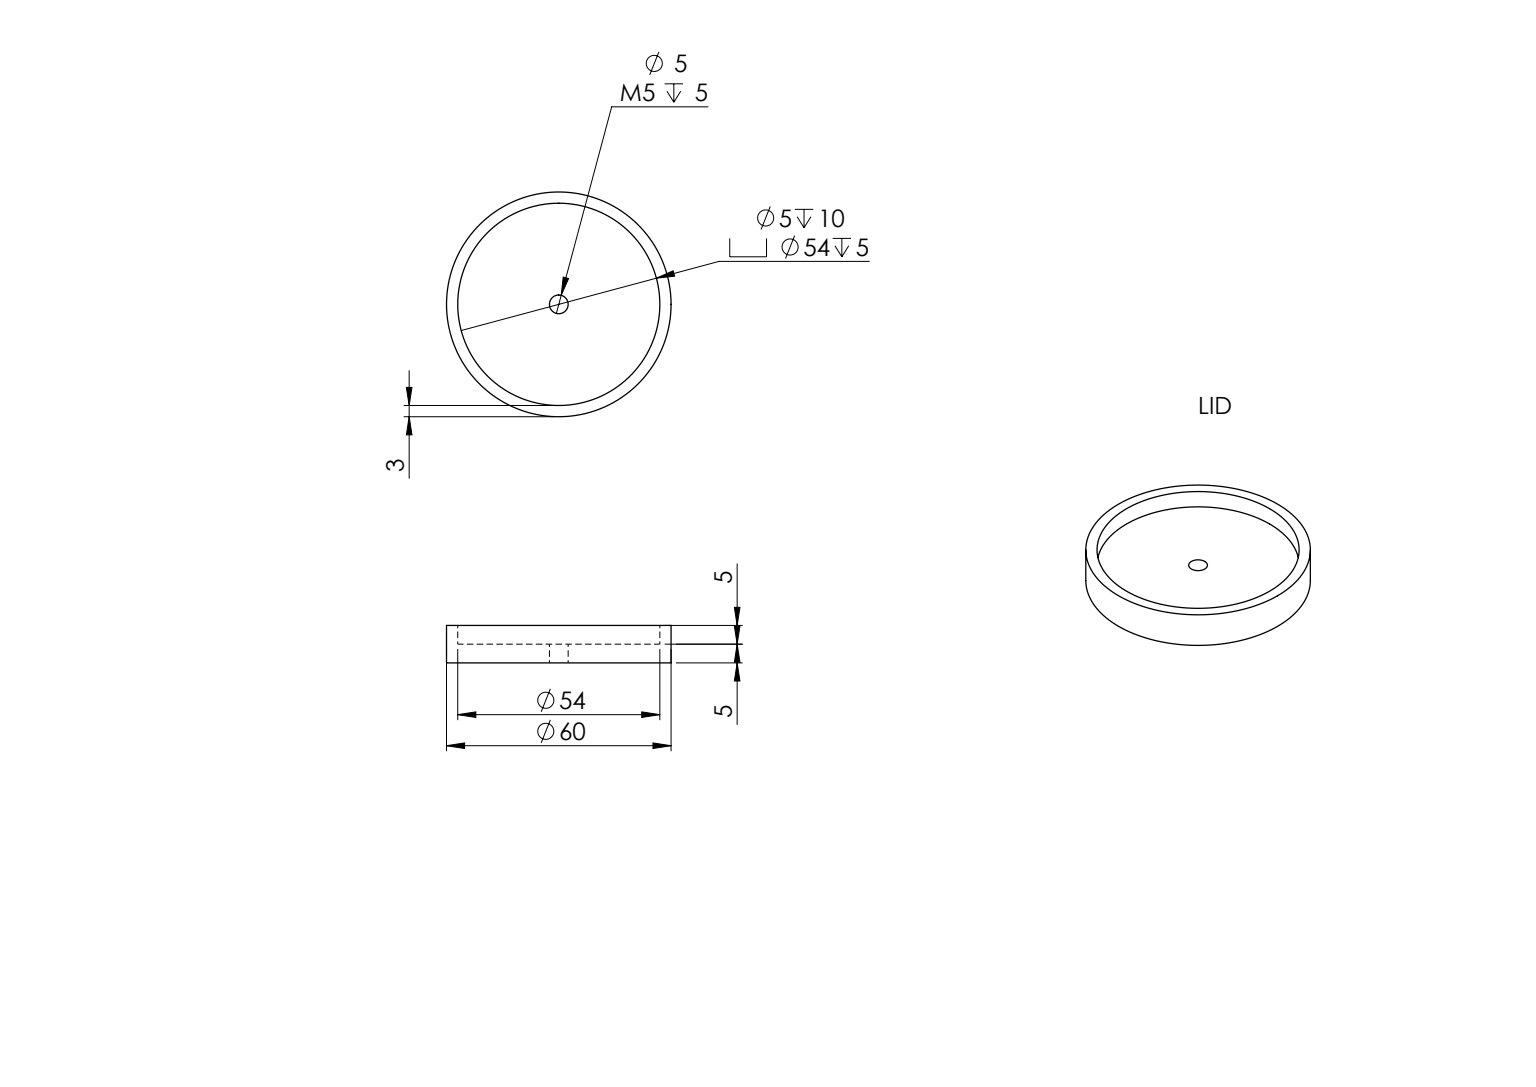
ISO-10303-21;
HEADER;
FILE_DESCRIPTION (('STEP AP214'),
    '1' );
FILE_NAME ('lid.step',
    '2026-10-24T15:06:47',
    ( '' ),
    ( '' ),
    'SwSTEP 2.0',
    'SolidWorks 2026',
    '' );
FILE_SCHEMA (( 'AUTOMOTIVE_DESIGN' ));
ENDSEC;

DATA;
#22=CYLINDRICAL_SURFACE ( 'NONE', #5038, 2.499999999999999556 ) ;
#32=CIRCLE ( 'NONE', #8383, 30.00000000000000000 ) ;
#64=AXIS2_PLACEMENT_3D ( 'NONE', #1231, #6667, #8456 ) ;
#84=VERTEX_POINT ( 'NONE', #3619 ) ;
#119=DIRECTION ( 'NONE',  ( -0.000000000000000000, -1.000000000000000000, -0.000000000000000000 ) ) ;
#144=AXIS2_PLACEMENT_3D ( 'NONE', #2203, #6849, #5404 ) ;
#246=ORIENTED_EDGE ( 'NONE', *, *, #1140, .T. ) ;
#259=CIRCLE ( 'NONE', #7786, 2.500000000000000000 ) ;
#260=CARTESIAN_POINT ( 'NONE',  ( 0.000000000000000000, 5.000000000000000000, -30.00000000000000000 ) ) ;
#274=CIRCLE ( 'NONE', #2111, 2.499999999999999556 ) ;
#365=CIRCLE ( 'NONE', #10244, 2.499999999999999556 ) ;
#377=ORIENTED_EDGE ( 'NONE', *, *, #7603, .T. ) ;
#411=PRODUCT_CONTEXT ( 'NONE', #6724, 'mechanical' ) ;
#447=CYLINDRICAL_SURFACE ( 'NONE', #8083, 27.00000000000000000 ) ;
#486=VERTEX_POINT ( 'NONE', #2361 ) ;
#492=CARTESIAN_POINT ( 'NONE',  ( 3.673940397442059178E-15, -5.000000000000000000, 30.00000000000000000 ) ) ;
#504=DIRECTION ( 'NONE',  ( 0.000000000000000000, 0.000000000000000000, -1.000000000000000000 ) ) ;
#529=FACE_BOUND ( 'NONE', #3018, .T. ) ;
#536=EDGE_LOOP ( 'NONE', ( #246, #377, #3425, #10307 ) ) ;
#556=FACE_OUTER_BOUND ( 'NONE', #3984, .T. ) ;
#564=DIRECTION ( 'NONE',  ( 0.000000000000000000, 0.000000000000000000, -1.000000000000000000 ) ) ;
#594=DIRECTION ( 'NONE',  ( 0.000000000000000000, 0.000000000000000000, -1.000000000000000000 ) ) ;
#618=DIRECTION ( 'NONE',  ( 0.000000000000000000, -1.000000000000000000, 0.000000000000000000 ) ) ;
#645=AXIS2_PLACEMENT_3D ( 'NONE', #7676, #618, #5331 ) ;
#718=DIRECTION ( 'NONE',  ( 0.000000000000000000, -1.000000000000000000, 0.000000000000000000 ) ) ;
#749=SHAPE_REPRESENTATION_RELATIONSHIP ( 'NONE' , 'NONE' ,  #2324, #4015 ) ;
#839=EDGE_CURVE ( 'NONE', #1713, #9182, #7041, .T. ) ;
#851=EDGE_LOOP ( 'NONE', ( #9977, #8377 ) ) ;
#934=EDGE_LOOP ( 'NONE', ( #1052, #10025 ) ) ;
#940=CIRCLE ( 'NONE', #3608, 27.00000000000000000 ) ;
#954=CIRCLE ( 'NONE', #7972, 30.00000000000000000 ) ;
#994=CARTESIAN_POINT ( 'NONE',  ( 0.000000000000000000, 5.000000000000000000, 0.000000000000000000 ) ) ;
#1044=FACE_OUTER_BOUND ( 'NONE', #3604, .T. ) ;
#1052=ORIENTED_EDGE ( 'NONE', *, *, #1402, .F. ) ;
#1094=DIRECTION ( 'NONE',  ( 0.000000000000000000, 0.000000000000000000, -1.000000000000000000 ) ) ;
#1121=EDGE_CURVE ( 'NONE', #3650, #2978, #9283, .T. ) ;
#1125=ORIENTED_EDGE ( 'NONE', *, *, #2957, .F. ) ;
#1126=DIRECTION ( 'NONE',  ( 0.000000000000000000, -1.000000000000000000, 0.000000000000000000 ) ) ;
#1140=EDGE_CURVE ( 'NONE', #1713, #7033, #8127, .T. ) ;
#1142=PRODUCT_DEFINITION ( 'UNKNOWN', '', #9806, #6436 ) ;
#1188=CYLINDRICAL_SURFACE ( 'NONE', #645, 27.00000000000000000 ) ;
#1194=EDGE_CURVE ( 'NONE', #84, #4497, #259, .T. ) ;
#1231=CARTESIAN_POINT ( 'NONE',  ( 0.000000000000000000, 0.000000000000000000, 0.000000000000000000 ) ) ;
#1253=EDGE_CURVE ( 'NONE', #2978, #3650, #940, .T. ) ;
#1310=FACE_OUTER_BOUND ( 'NONE', #8227, .T. ) ;
#1375=CARTESIAN_POINT ( 'NONE',  ( 0.000000000000000000, 5.000000000000000000, 0.000000000000000000 ) ) ;
#1402=EDGE_CURVE ( 'NONE', #4497, #84, #2382, .T. ) ;
#1419=CARTESIAN_POINT ( 'NONE',  ( 3.673940397442059178E-15, 5.000000000000000000, 30.00000000000000000 ) ) ;
#1448=PLANE ( 'NONE',  #2297 ) ;
#1451=CARTESIAN_POINT ( 'NONE',  ( 0.000000000000000000, 5.000000000000000000, 0.000000000000000000 ) ) ;
#1466=CARTESIAN_POINT ( 'NONE',  ( 0.000000000000000000, 0.000000000000000000, -27.00000000000000000 ) ) ;
#1472=DIRECTION ( 'NONE',  ( 0.000000000000000000, -0.000000000000000000, -1.000000000000000000 ) ) ;
#1483=VECTOR ( 'NONE', #6999, 1000.000000000000000 ) ;
#1492=LINE ( 'NONE', #4577, #6566 ) ;
#1531=DIRECTION ( 'NONE',  ( 0.000000000000000000, 0.000000000000000000, -1.000000000000000000 ) ) ;
#1649=DIRECTION ( 'NONE',  ( 0.000000000000000000, 0.000000000000000000, -1.000000000000000000 ) ) ;
#1713=VERTEX_POINT ( 'NONE', #260 ) ;
#1755=ADVANCED_FACE ( 'NONE', ( #1044 ), #4967, .T. ) ;
#1801=LINE ( 'NONE', #6571, #2147 ) ;
#1982=DIRECTION ( 'NONE',  ( 0.000000000000000000, 0.000000000000000000, -1.000000000000000000 ) ) ;
#2018=AXIS2_PLACEMENT_3D ( 'NONE', #3168, #119, #3215 ) ;
#2041=EDGE_CURVE ( 'NONE', #486, #7555, #365, .T. ) ;
#2111=AXIS2_PLACEMENT_3D ( 'NONE', #9162, #4559, #1982 ) ;
#2116=ADVANCED_FACE ( 'NONE', ( #3957 ), #22, .F. ) ;
#2120=DIRECTION ( 'NONE',  ( 0.000000000000000000, -1.000000000000000000, 0.000000000000000000 ) ) ;
#2147=VECTOR ( 'NONE', #8884, 1000.000000000000000 ) ;
#2148=DIRECTION ( 'NONE',  ( 0.000000000000000000, -0.000000000000000000, -1.000000000000000000 ) ) ;
#2188=CYLINDRICAL_SURFACE ( 'NONE', #6682, 2.499999999999999556 ) ;
#2194=ORIENTED_EDGE ( 'NONE', *, *, #7603, .F. ) ;
#2203=CARTESIAN_POINT ( 'NONE',  ( 0.000000000000000000, -5.000000000000000000, 0.000000000000000000 ) ) ;
#2235=MECHANICAL_DESIGN_GEOMETRIC_PRESENTATION_REPRESENTATION('',(#6248),#7465);
#2244=CARTESIAN_POINT ( 'NONE',  ( 0.000000000000000000, 5.000000000000000000, -27.00000000000000000 ) ) ;
#2297=AXIS2_PLACEMENT_3D ( 'NONE', #4641, #2120, #7834 ) ;
#2324=SHAPE_REPRESENTATION ( 'lid', ( #5055 ), #7565 ) ;
#2349=ORIENTED_EDGE ( 'NONE', *, *, #3197, .T. ) ;
#2361=CARTESIAN_POINT ( 'NONE',  ( 3.061616997868382648E-16, 0.000000000000000000, 2.499999999999999556 ) ) ;
#2382=CIRCLE ( 'NONE', #2018, 2.500000000000000000 ) ;
#2419=SURFACE_SIDE_STYLE ('',( #7075 ) ) ;
#2519=DIRECTION ( 'NONE',  ( 0.000000000000000000, -1.000000000000000000, 0.000000000000000000 ) ) ;
#2587=ORIENTED_EDGE ( 'NONE', *, *, #8719, .T. ) ;
#2786=DIRECTION ( 'NONE',  ( 0.000000000000000000, 0.000000000000000000, -1.000000000000000000 ) ) ;
#2790=CLOSED_SHELL ( 'NONE', ( #2116, #10132, #5453, #1755, #9213, #7285, #7034, #7008, #6121 ) ) ;
#2899=MECHANICAL_DESIGN_GEOMETRIC_PRESENTATION_REPRESENTATION('',(#7077),#4740);
#2922=FACE_OUTER_BOUND ( 'NONE', #4194, .T. ) ;
#2957=EDGE_CURVE ( 'NONE', #4542, #4452, #6719, .T. ) ;
#2978=VERTEX_POINT ( 'NONE', #8014 ) ;
#3018=EDGE_LOOP ( 'NONE', ( #5288, #5280 ) ) ;
#3095=ORIENTED_EDGE ( 'NONE', *, *, #1253, .F. ) ;
#3117=CARTESIAN_POINT ( 'NONE',  ( 0.000000000000000000, -5.000000000000000000, 0.000000000000000000 ) ) ;
#3145=ORIENTED_EDGE ( 'NONE', *, *, #3853, .F. ) ;
#3159=AXIS2_PLACEMENT_3D ( 'NONE', #5347, #8424, #1472 ) ;
#3168=CARTESIAN_POINT ( 'NONE',  ( 0.000000000000000000, -5.000000000000000000, 0.000000000000000000 ) ) ;
#3197=EDGE_CURVE ( 'NONE', #7555, #4497, #1492, .T. ) ;
#3204=DIRECTION ( 'NONE',  ( 0.000000000000000000, 0.000000000000000000, -1.000000000000000000 ) ) ;
#3215=DIRECTION ( 'NONE',  ( 0.000000000000000000, 0.000000000000000000, -1.000000000000000000 ) ) ;
#3291=( NAMED_UNIT ( * ) SI_UNIT ( $, .STERADIAN. ) SOLID_ANGLE_UNIT ( ) );
#3425=ORIENTED_EDGE ( 'NONE', *, *, #9123, .F. ) ;
#3514=DIRECTION ( 'NONE',  ( 0.000000000000000000, -1.000000000000000000, 0.000000000000000000 ) ) ;
#3548=ORIENTED_EDGE ( 'NONE', *, *, #3197, .F. ) ;
#3557=EDGE_CURVE ( 'NONE', #7033, #1713, #32, .T. ) ;
#3604=EDGE_LOOP ( 'NONE', ( #2194, #4615, #9752, #6085 ) ) ;
#3608=AXIS2_PLACEMENT_3D ( 'NONE', #1375, #4568, #1531 ) ;
#3619=CARTESIAN_POINT ( 'NONE',  ( 3.061616997868383141E-16, -5.000000000000000000, 2.500000000000000000 ) ) ;
#3650=VERTEX_POINT ( 'NONE', #6564 ) ;
#3720=UNCERTAINTY_MEASURE_WITH_UNIT (LENGTH_MEASURE( 1.000000000000000082E-05 ), #9441, 'distance_accuracy_value', 'NONE');
#3736=ORIENTED_EDGE ( 'NONE', *, *, #1402, .T. ) ;
#3741=LINE ( 'NONE', #6923, #8462 ) ;
#3759=CARTESIAN_POINT ( 'NONE',  ( 0.000000000000000000, -5.000000000000000000, 0.000000000000000000 ) ) ;
#3853=EDGE_CURVE ( 'NONE', #486, #84, #7440, .T. ) ;
#3887=( NAMED_UNIT ( * ) PLANE_ANGLE_UNIT ( ) SI_UNIT ( $, .RADIAN. ) );
#3913=DIRECTION ( 'NONE',  ( 1.000000000000000000, 0.000000000000000000, 0.000000000000000000 ) ) ;
#3957=FACE_OUTER_BOUND ( 'NONE', #8668, .T. ) ;
#3984=EDGE_LOOP ( 'NONE', ( #9941, #4463 ) ) ;
#3989=AXIS2_PLACEMENT_3D ( 'NONE', #4608, #7801, #2148 ) ;
#3995=SURFACE_STYLE_USAGE ( .BOTH. , #2419 ) ;
#4015=ADVANCED_BREP_SHAPE_REPRESENTATION ( '', ( #9927, #5055 ), #7565 ) ;
#4092=FILL_AREA_STYLE ('',( #9587 ) ) ;
#4154=DIRECTION ( 'NONE',  ( 0.000000000000000000, 0.000000000000000000, 1.000000000000000000 ) ) ;
#4194=EDGE_LOOP ( 'NONE', ( #4343, #3095, #4575, #9751 ) ) ;
#4301=DIRECTION ( 'NONE',  ( 0.000000000000000000, -1.000000000000000000, 0.000000000000000000 ) ) ;
#4343=ORIENTED_EDGE ( 'NONE', *, *, #8719, .F. ) ;
#4388=SHAPE_DEFINITION_REPRESENTATION ( #9536, #2324 ) ;
#4446=PLANE ( 'NONE',  #3989 ) ;
#4452=VERTEX_POINT ( 'NONE', #9778 ) ;
#4463=ORIENTED_EDGE ( 'NONE', *, *, #3557, .F. ) ;
#4497=VERTEX_POINT ( 'NONE', #6684 ) ;
#4511=DIRECTION ( 'NONE',  ( -0.000000000000000000, -1.000000000000000000, -0.000000000000000000 ) ) ;
#4516=ORIENTED_EDGE ( 'NONE', *, *, #1121, .F. ) ;
#4542=VERTEX_POINT ( 'NONE', #1466 ) ;
#4559=DIRECTION ( 'NONE',  ( -0.000000000000000000, -1.000000000000000000, -0.000000000000000000 ) ) ;
#4568=DIRECTION ( 'NONE',  ( 0.000000000000000000, -1.000000000000000000, 0.000000000000000000 ) ) ;
#4575=ORIENTED_EDGE ( 'NONE', *, *, #7297, .T. ) ;
#4577=CARTESIAN_POINT ( 'NONE',  ( 0.000000000000000000, -5.000000000000000000, -2.499999999999999556 ) ) ;
#4600=APPLICATION_CONTEXT ( 'automotive_design' ) ;
#4608=CARTESIAN_POINT ( 'NONE',  ( 0.000000000000000000, 0.000000000000000000, 0.000000000000000000 ) ) ;
#4615=ORIENTED_EDGE ( 'NONE', *, *, #3557, .T. ) ;
#4641=CARTESIAN_POINT ( 'NONE',  ( 0.000000000000000000, 5.000000000000000000, 0.000000000000000000 ) ) ;
#4652=EDGE_LOOP ( 'NONE', ( #4516, #2587, #5419, #6353 ) ) ;
#4740=( GEOMETRIC_REPRESENTATION_CONTEXT ( 3 ) GLOBAL_UNCERTAINTY_ASSIGNED_CONTEXT ( ( #5402 ) ) GLOBAL_UNIT_ASSIGNED_CONTEXT ( ( #9623, #4862, #3291 ) ) REPRESENTATION_CONTEXT ( 'NONE', 'WORKASPACE' ) );
#4760=UNCERTAINTY_MEASURE_WITH_UNIT (LENGTH_MEASURE( 1.000000000000000082E-05 ), #6296, 'distance_accuracy_value', 'NONE');
#4787=DIRECTION ( 'NONE',  ( -0.000000000000000000, -1.000000000000000000, -0.000000000000000000 ) ) ;
#4862=( NAMED_UNIT ( * ) PLANE_ANGLE_UNIT ( ) SI_UNIT ( $, .RADIAN. ) );
#4936=DIRECTION ( 'NONE',  ( -0.000000000000000000, -1.000000000000000000, -0.000000000000000000 ) ) ;
#4967=CYLINDRICAL_SURFACE ( 'NONE', #9724, 30.00000000000000000 ) ;
#5038=AXIS2_PLACEMENT_3D ( 'NONE', #7984, #4936, #1649 ) ;
#5055=AXIS2_PLACEMENT_3D ( 'NONE', #9842, #4154, #9744 ) ;
#5192=DIRECTION ( 'NONE',  ( 0.000000000000000000, -1.000000000000000000, 0.000000000000000000 ) ) ;
#5237=CARTESIAN_POINT ( 'NONE',  ( 0.000000000000000000, 5.000000000000000000, 0.000000000000000000 ) ) ;
#5248=DIRECTION ( 'NONE',  ( -0.000000000000000000, -1.000000000000000000, -0.000000000000000000 ) ) ;
#5255=DIRECTION ( 'NONE',  ( 0.000000000000000000, 0.000000000000000000, -1.000000000000000000 ) ) ;
#5280=ORIENTED_EDGE ( 'NONE', *, *, #2041, .T. ) ;
#5284=FACE_OUTER_BOUND ( 'NONE', #851, .T. ) ;
#5288=ORIENTED_EDGE ( 'NONE', *, *, #8840, .T. ) ;
#5331=DIRECTION ( 'NONE',  ( 0.000000000000000000, 0.000000000000000000, -1.000000000000000000 ) ) ;
#5347=CARTESIAN_POINT ( 'NONE',  ( 0.000000000000000000, -5.000000000000000000, 0.000000000000000000 ) ) ;
#5402=UNCERTAINTY_MEASURE_WITH_UNIT (LENGTH_MEASURE( 1.000000000000000082E-05 ), #9623, 'distance_accuracy_value', 'NONE');
#5404=DIRECTION ( 'NONE',  ( 0.000000000000000000, 0.000000000000000000, -1.000000000000000000 ) ) ;
#5419=ORIENTED_EDGE ( 'NONE', *, *, #10119, .T. ) ;
#5436=FACE_BOUND ( 'NONE', #9392, .T. ) ;
#5453=ADVANCED_FACE ( 'NONE', ( #10201 ), #9411, .T. ) ;
#5613=ORIENTED_EDGE ( 'NONE', *, *, #3853, .T. ) ;
#5905=DIRECTION ( 'NONE',  ( 0.000000000000000000, -1.000000000000000000, 0.000000000000000000 ) ) ;
#6085=ORIENTED_EDGE ( 'NONE', *, *, #6915, .F. ) ;
#6105=LINE ( 'NONE', #2244, #1483 ) ;
#6121=ADVANCED_FACE ( 'NONE', ( #9144 ), #2188, .F. ) ;
#6207=CARTESIAN_POINT ( 'NONE',  ( 0.000000000000000000, -5.000000000000000000, -30.00000000000000000 ) ) ;
#6231=PLANE ( 'NONE',  #3159 ) ;
#6240=( NAMED_UNIT ( * ) PLANE_ANGLE_UNIT ( ) SI_UNIT ( $, .RADIAN. ) );
#6248=STYLED_ITEM ( 'NONE', ( #8071 ), #4015 ) ;
#6296=( LENGTH_UNIT ( ) NAMED_UNIT ( * ) SI_UNIT ( .MILLI., .METRE. ) );
#6317=DIRECTION ( 'NONE',  ( 0.000000000000000000, -1.000000000000000000, 0.000000000000000000 ) ) ;
#6353=ORIENTED_EDGE ( 'NONE', *, *, #7297, .F. ) ;
#6397=( NAMED_UNIT ( * ) SI_UNIT ( $, .STERADIAN. ) SOLID_ANGLE_UNIT ( ) );
#6436=PRODUCT_DEFINITION_CONTEXT ( 'detailed design', #4600, 'design' ) ;
#6526=ORIENTED_EDGE ( 'NONE', *, *, #1253, .T. ) ;
#6564=CARTESIAN_POINT ( 'NONE',  ( 3.306546357697853733E-15, 5.000000000000000000, 27.00000000000000000 ) ) ;
#6566=VECTOR ( 'NONE', #5248, 1000.000000000000000 ) ;
#6567=CIRCLE ( 'NONE', #64, 27.00000000000000000 ) ;
#6571=CARTESIAN_POINT ( 'NONE',  ( 3.673940397442059178E-15, 5.000000000000000000, 30.00000000000000000 ) ) ;
#6667=DIRECTION ( 'NONE',  ( 0.000000000000000000, -1.000000000000000000, 0.000000000000000000 ) ) ;
#6682=AXIS2_PLACEMENT_3D ( 'NONE', #3759, #9237, #8464 ) ;
#6684=CARTESIAN_POINT ( 'NONE',  ( 0.000000000000000000, -5.000000000000000000, -2.500000000000000000 ) ) ;
#6719=CIRCLE ( 'NONE', #8230, 27.00000000000000000 ) ;
#6724=APPLICATION_CONTEXT ( 'automotive_design' ) ;
#6730=COLOUR_RGB ( '',0.8941176470588234615, 0.8941176470588234615, 0.8941176470588234615 ) ;
#6849=DIRECTION ( 'NONE',  ( 0.000000000000000000, -1.000000000000000000, 0.000000000000000000 ) ) ;
#6875=VECTOR ( 'NONE', #10013, 1000.000000000000000 ) ;
#6915=EDGE_CURVE ( 'NONE', #8764, #9182, #8494, .T. ) ;
#6923=CARTESIAN_POINT ( 'NONE',  ( 3.306546357697853733E-15, 5.000000000000000000, 27.00000000000000000 ) ) ;
#6987=CARTESIAN_POINT ( 'NONE',  ( 0.000000000000000000, 5.000000000000000000, -30.00000000000000000 ) ) ;
#6999=DIRECTION ( 'NONE',  ( 0.000000000000000000, -1.000000000000000000, 0.000000000000000000 ) ) ;
#7008=ADVANCED_FACE ( 'NONE', ( #8536, #5284 ), #6231, .T. ) ;
#7033=VERTEX_POINT ( 'NONE', #1419 ) ;
#7034=ADVANCED_FACE ( 'NONE', ( #529, #1310 ), #4446, .F. ) ;
#7041=LINE ( 'NONE', #6987, #9955 ) ;
#7075=SURFACE_STYLE_FILL_AREA ( #4092 ) ;
#7077=STYLED_ITEM('',(#10387),#9927);
#7093=ORIENTED_EDGE ( 'NONE', *, *, #1121, .T. ) ;
#7285=ADVANCED_FACE ( 'NONE', ( #2922 ), #1188, .F. ) ;
#7297=EDGE_CURVE ( 'NONE', #2978, #4542, #6105, .T. ) ;
#7352=CARTESIAN_POINT ( 'NONE',  ( 0.000000000000000000, 0.000000000000000000, -2.499999999999999556 ) ) ;
#7440=LINE ( 'NONE', #7659, #6875 ) ;
#7458=ORIENTED_EDGE ( 'NONE', *, *, #2041, .F. ) ;
#7465=( GEOMETRIC_REPRESENTATION_CONTEXT ( 3 ) GLOBAL_UNCERTAINTY_ASSIGNED_CONTEXT ( ( #4760 ) ) GLOBAL_UNIT_ASSIGNED_CONTEXT ( ( #6296, #6240, #8022 ) ) REPRESENTATION_CONTEXT ( 'NONE', 'WORKASPACE' ) );
#7503=CARTESIAN_POINT ( 'NONE',  ( 0.000000000000000000, 5.000000000000000000, 0.000000000000000000 ) ) ;
#7555=VERTEX_POINT ( 'NONE', #7352 ) ;
#7565=( GEOMETRIC_REPRESENTATION_CONTEXT ( 3 ) GLOBAL_UNCERTAINTY_ASSIGNED_CONTEXT ( ( #3720 ) ) GLOBAL_UNIT_ASSIGNED_CONTEXT ( ( #9441, #3887, #6397 ) ) REPRESENTATION_CONTEXT ( 'NONE', 'WORKASPACE' ) );
#7603=EDGE_CURVE ( 'NONE', #7033, #8764, #1801, .T. ) ;
#7649=DIRECTION ( 'NONE',  ( 1.000000000000000000, 0.000000000000000000, 0.000000000000000000 ) ) ;
#7659=CARTESIAN_POINT ( 'NONE',  ( 3.061616997868382648E-16, -5.000000000000000000, 2.499999999999999556 ) ) ;
#7673=DIRECTION ( 'NONE',  ( 0.000000000000000000, -1.000000000000000000, 0.000000000000000000 ) ) ;
#7676=CARTESIAN_POINT ( 'NONE',  ( 0.000000000000000000, 5.000000000000000000, 0.000000000000000000 ) ) ;
#7778=DIRECTION ( 'NONE',  ( 0.000000000000000000, -1.000000000000000000, 0.000000000000000000 ) ) ;
#7782=AXIS2_PLACEMENT_3D ( 'NONE', #8518, #7673, #564 ) ;
#7786=AXIS2_PLACEMENT_3D ( 'NONE', #3117, #4511, #594 ) ;
#7801=DIRECTION ( 'NONE',  ( 0.000000000000000000, -1.000000000000000000, 0.000000000000000000 ) ) ;
#7834=DIRECTION ( 'NONE',  ( 0.000000000000000000, -0.000000000000000000, -1.000000000000000000 ) ) ;
#7931=CARTESIAN_POINT ( 'NONE',  ( 0.000000000000000000, 0.000000000000000000, 0.000000000000000000 ) ) ;
#7972=AXIS2_PLACEMENT_3D ( 'NONE', #9229, #7778, #5255 ) ;
#7984=CARTESIAN_POINT ( 'NONE',  ( 0.000000000000000000, -5.000000000000000000, 0.000000000000000000 ) ) ;
#8014=CARTESIAN_POINT ( 'NONE',  ( 0.000000000000000000, 5.000000000000000000, -27.00000000000000000 ) ) ;
#8022=( NAMED_UNIT ( * ) SI_UNIT ( $, .STERADIAN. ) SOLID_ANGLE_UNIT ( ) );
#8071=PRESENTATION_STYLE_ASSIGNMENT (( #3995 ) ) ;
#8083=AXIS2_PLACEMENT_3D ( 'NONE', #7503, #1126, #504 ) ;
#8127=CIRCLE ( 'NONE', #8795, 30.00000000000000000 ) ;
#8159=CARTESIAN_POINT ( 'NONE',  ( 0.000000000000000000, 0.000000000000000000, 0.000000000000000000 ) ) ;
#8227=EDGE_LOOP ( 'NONE', ( #1125, #9020 ) ) ;
#8230=AXIS2_PLACEMENT_3D ( 'NONE', #8159, #2519, #3204 ) ;
#8272=ORIENTED_EDGE ( 'NONE', *, *, #8840, .F. ) ;
#8377=ORIENTED_EDGE ( 'NONE', *, *, #6915, .T. ) ;
#8383=AXIS2_PLACEMENT_3D ( 'NONE', #1451, #718, #3913 ) ;
#8424=DIRECTION ( 'NONE',  ( 0.000000000000000000, -1.000000000000000000, 0.000000000000000000 ) ) ;
#8456=DIRECTION ( 'NONE',  ( 0.000000000000000000, 0.000000000000000000, -1.000000000000000000 ) ) ;
#8462=VECTOR ( 'NONE', #5192, 1000.000000000000000 ) ;
#8464=DIRECTION ( 'NONE',  ( 0.000000000000000000, 0.000000000000000000, -1.000000000000000000 ) ) ;
#8494=CIRCLE ( 'NONE', #144, 30.00000000000000000 ) ;
#8518=CARTESIAN_POINT ( 'NONE',  ( 0.000000000000000000, 5.000000000000000000, 0.000000000000000000 ) ) ;
#8527=ORIENTED_EDGE ( 'NONE', *, *, #1194, .T. ) ;
#8536=FACE_BOUND ( 'NONE', #934, .T. ) ;
#8635=AXIS2_PLACEMENT_3D ( 'NONE', #9215, #3514, #2786 ) ;
#8668=EDGE_LOOP ( 'NONE', ( #7458, #5613, #8527, #3548 ) ) ;
#8719=EDGE_CURVE ( 'NONE', #3650, #4452, #3741, .T. ) ;
#8764=VERTEX_POINT ( 'NONE', #492 ) ;
#8779=PRODUCT ( 'lid', 'lid', '', ( #411 ) ) ;
#8795=AXIS2_PLACEMENT_3D ( 'NONE', #5237, #4301, #7649 ) ;
#8840=EDGE_CURVE ( 'NONE', #7555, #486, #274, .T. ) ;
#8884=DIRECTION ( 'NONE',  ( 0.000000000000000000, -1.000000000000000000, 0.000000000000000000 ) ) ;
#9020=ORIENTED_EDGE ( 'NONE', *, *, #10119, .F. ) ;
#9123=EDGE_CURVE ( 'NONE', #9182, #8764, #954, .T. ) ;
#9144=FACE_OUTER_BOUND ( 'NONE', #9800, .T. ) ;
#9162=CARTESIAN_POINT ( 'NONE',  ( 0.000000000000000000, 0.000000000000000000, 0.000000000000000000 ) ) ;
#9182=VERTEX_POINT ( 'NONE', #6207 ) ;
#9213=ADVANCED_FACE ( 'NONE', ( #5436, #556 ), #1448, .F. ) ;
#9215=CARTESIAN_POINT ( 'NONE',  ( 0.000000000000000000, 5.000000000000000000, 0.000000000000000000 ) ) ;
#9229=CARTESIAN_POINT ( 'NONE',  ( 0.000000000000000000, -5.000000000000000000, 0.000000000000000000 ) ) ;
#9237=DIRECTION ( 'NONE',  ( -0.000000000000000000, -1.000000000000000000, -0.000000000000000000 ) ) ;
#9283=CIRCLE ( 'NONE', #8635, 27.00000000000000000 ) ;
#9392=EDGE_LOOP ( 'NONE', ( #6526, #7093 ) ) ;
#9411=CYLINDRICAL_SURFACE ( 'NONE', #7782, 30.00000000000000000 ) ;
#9441=( LENGTH_UNIT ( ) NAMED_UNIT ( * ) SI_UNIT ( .MILLI., .METRE. ) );
#9509=DIRECTION ( 'NONE',  ( 0.000000000000000000, 0.000000000000000000, -1.000000000000000000 ) ) ;
#9536=PRODUCT_DEFINITION_SHAPE ( 'NONE', 'NONE',  #1142 ) ;
#9587=FILL_AREA_STYLE_COLOUR ( '', #6730 ) ;
#9623=( LENGTH_UNIT ( ) NAMED_UNIT ( * ) SI_UNIT ( .MILLI., .METRE. ) );
#9724=AXIS2_PLACEMENT_3D ( 'NONE', #994, #5905, #1094 ) ;
#9744=DIRECTION ( 'NONE',  ( 1.000000000000000000, 0.000000000000000000, 0.000000000000000000 ) ) ;
#9751=ORIENTED_EDGE ( 'NONE', *, *, #2957, .T. ) ;
#9752=ORIENTED_EDGE ( 'NONE', *, *, #839, .T. ) ;
#9778=CARTESIAN_POINT ( 'NONE',  ( 3.306546357697853733E-15, 0.000000000000000000, 27.00000000000000000 ) ) ;
#9800=EDGE_LOOP ( 'NONE', ( #3145, #8272, #2349, #3736 ) ) ;
#9806=PRODUCT_DEFINITION_FORMATION_WITH_SPECIFIED_SOURCE ( 'ANY', '', #8779, .NOT_KNOWN. ) ;
#9842=CARTESIAN_POINT ( 'NONE',  ( 0.000000000000000000, 0.000000000000000000, 0.000000000000000000 ) ) ;
#9927=MANIFOLD_SOLID_BREP ( 'AdvancedHole1', #2790 ) ;
#9941=ORIENTED_EDGE ( 'NONE', *, *, #1140, .F. ) ;
#9955=VECTOR ( 'NONE', #6317, 1000.000000000000000 ) ;
#9972=FACE_OUTER_BOUND ( 'NONE', #4652, .T. ) ;
#9977=ORIENTED_EDGE ( 'NONE', *, *, #9123, .T. ) ;
#10013=DIRECTION ( 'NONE',  ( -0.000000000000000000, -1.000000000000000000, -0.000000000000000000 ) ) ;
#10025=ORIENTED_EDGE ( 'NONE', *, *, #1194, .F. ) ;
#10119=EDGE_CURVE ( 'NONE', #4452, #4542, #6567, .T. ) ;
#10132=ADVANCED_FACE ( 'NONE', ( #9972 ), #447, .F. ) ;
#10201=FACE_OUTER_BOUND ( 'NONE', #536, .T. ) ;
#10244=AXIS2_PLACEMENT_3D ( 'NONE', #7931, #4787, #9509 ) ;
#10307=ORIENTED_EDGE ( 'NONE', *, *, #839, .F. ) ;
#10381=COLOUR_RGB('Light Blue',0.38,0.62,0.78);
#10382=FILL_AREA_STYLE_COLOUR('',#10381);
#10383=FILL_AREA_STYLE('',(#10382));
#10384=SURFACE_STYLE_FILL_AREA(#10383);
#10385=SURFACE_SIDE_STYLE('',(#10384));
#10386=SURFACE_STYLE_USAGE(.BOTH.,#10385);
#10387=PRESENTATION_STYLE_ASSIGNMENT((#10386));
ENDSEC;
END-ISO-10303-21;
